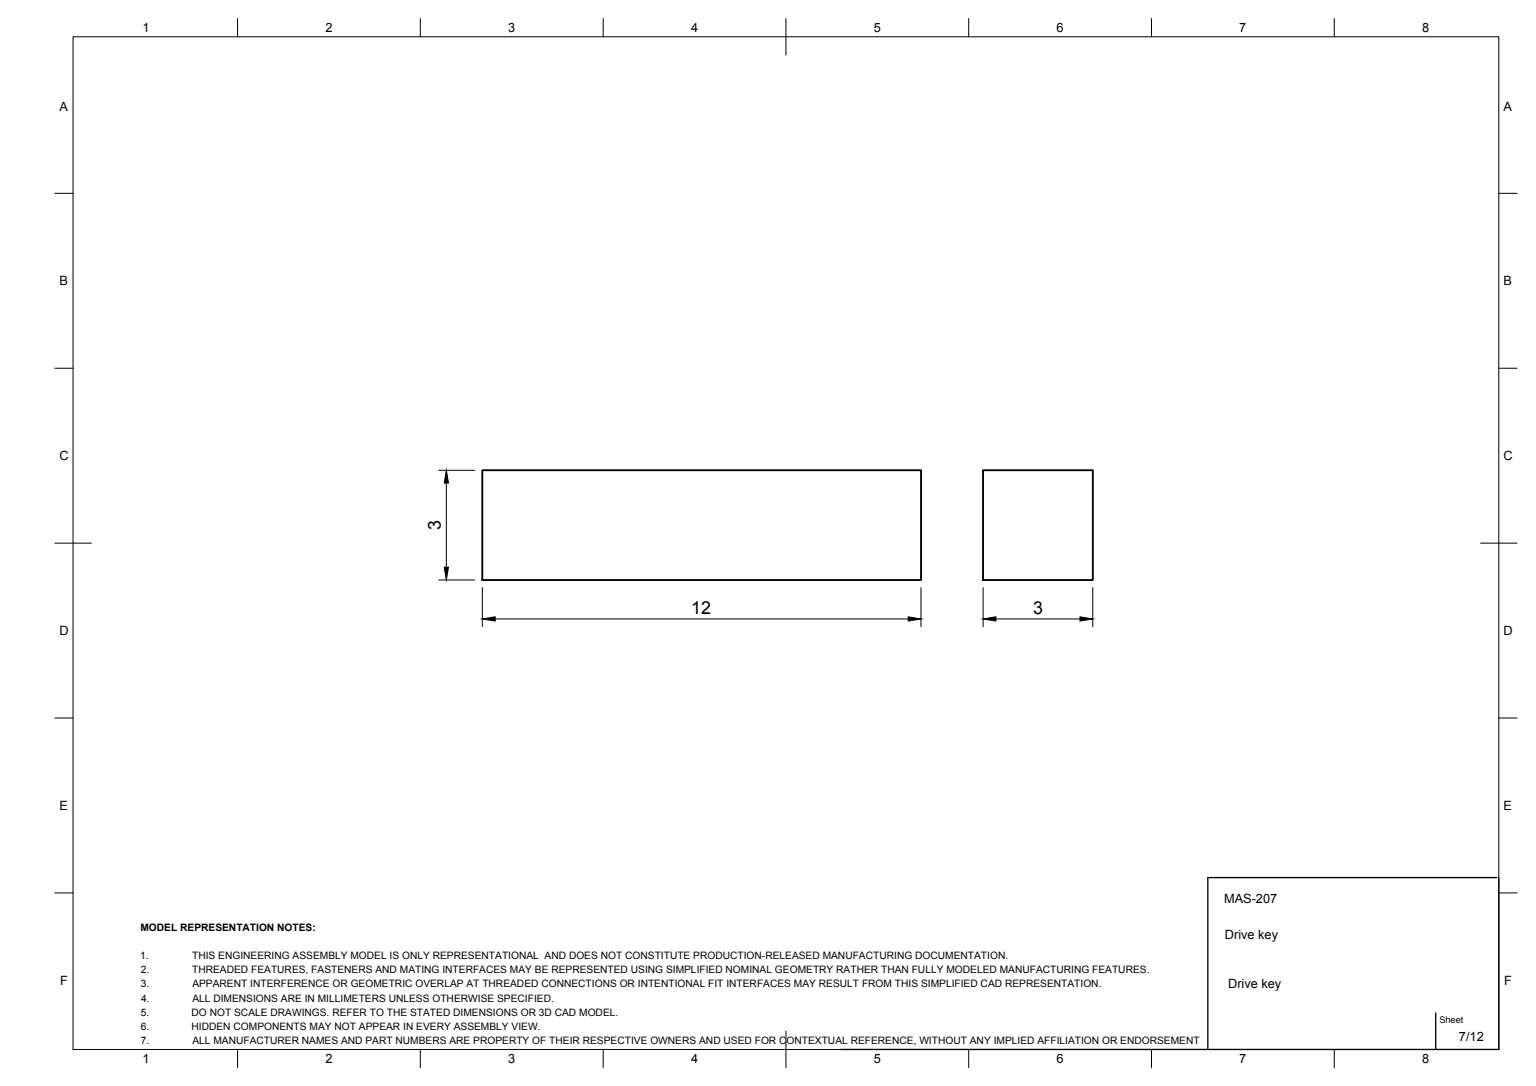
ISO-10303-21;
HEADER;
/* Generated by software containing ST-Developer
 * from STEP Tools, Inc. (www.steptools.com) 
 */

FILE_DESCRIPTION(
/* description */ ('Independent six-slot Geneva indexer. Center distance100, drive radius
50, 60degree indexing per input revolution with120degree engagement an
d240degree dwell. Native machined concave locking faces and relieved d
isk; replaceable retained drive pin; keyed output shaft. Geometry traj
ectory checks use calculated indexing positions, not a contact-dynamic
s simulation. No load or production rating assigned.'),
/* implementation_level */ '2;1');

FILE_NAME(
/* name */ 'Drive key.step',
/* time_stamp */ '2026-11-09T17:53:22-08:00',
/* author */ (''),
/* organization */ (''),
/* preprocessor_version */ 'ST-DEVELOPER v20.2',
/* originating_system */ 'Autodesk Translation Framework v15.17.0.0',
/* authorisation */ '');

FILE_SCHEMA (('AUTOMOTIVE_DESIGN { 1 0 10303 214 3 1 1 }'));
ENDSEC;

DATA;
#10=MECHANICAL_DESIGN_GEOMETRIC_PRESENTATION_REPRESENTATION('',(#105),#4149);
#83=SHAPE_REPRESENTATION_RELATIONSHIP('SRR','None',#4200,#94);
#94=ADVANCED_BREP_SHAPE_REPRESENTATION('',(#116),#4142);
#105=STYLED_ITEM('',(#4264),#116);
#116=MANIFOLD_SOLID_BREP('Body1',#2299);
#213=PLANE('',#2621);
#214=PLANE('',#2622);
#215=PLANE('',#2623);
#216=PLANE('',#2624);
#217=PLANE('',#2625);
#218=PLANE('',#2626);
#333=FACE_OUTER_BOUND('',#494,.T.);
#334=FACE_OUTER_BOUND('',#495,.T.);
#335=FACE_OUTER_BOUND('',#496,.T.);
#336=FACE_OUTER_BOUND('',#497,.T.);
#337=FACE_OUTER_BOUND('',#498,.T.);
#338=FACE_OUTER_BOUND('',#499,.T.);
#494=EDGE_LOOP('',(#1968,#1969,#1970,#1971));
#495=EDGE_LOOP('',(#1972,#1973,#1974,#1975));
#496=EDGE_LOOP('',(#1976,#1977,#1978,#1979));
#497=EDGE_LOOP('',(#1980,#1981,#1982,#1983));
#498=EDGE_LOOP('',(#1984,#1985,#1986,#1987));
#499=EDGE_LOOP('',(#1988,#1989,#1990,#1991));
#686=LINE('',#3953,#858);
#687=LINE('',#3955,#859);
#688=LINE('',#3957,#860);
#689=LINE('',#3958,#861);
#690=LINE('',#3961,#862);
#691=LINE('',#3963,#863);
#692=LINE('',#3964,#864);
#693=LINE('',#3967,#865);
#694=LINE('',#3969,#866);
#695=LINE('',#3970,#867);
#696=LINE('',#3972,#868);
#697=LINE('',#3973,#869);
#858=VECTOR('',#3243,10.);
#859=VECTOR('',#3244,10.);
#860=VECTOR('',#3245,10.);
#861=VECTOR('',#3246,10.);
#862=VECTOR('',#3249,10.);
#863=VECTOR('',#3250,10.);
#864=VECTOR('',#3251,10.);
#865=VECTOR('',#3254,10.);
#866=VECTOR('',#3255,10.);
#867=VECTOR('',#3256,10.);
#868=VECTOR('',#3259,10.);
#869=VECTOR('',#3260,10.);
#1168=VERTEX_POINT('',#3951);
#1169=VERTEX_POINT('',#3952);
#1170=VERTEX_POINT('',#3954);
#1171=VERTEX_POINT('',#3956);
#1172=VERTEX_POINT('',#3960);
#1173=VERTEX_POINT('',#3962);
#1174=VERTEX_POINT('',#3966);
#1175=VERTEX_POINT('',#3968);
#1442=EDGE_CURVE('',#1168,#1169,#686,.T.);
#1443=EDGE_CURVE('',#1169,#1170,#687,.T.);
#1444=EDGE_CURVE('',#1171,#1170,#688,.T.);
#1445=EDGE_CURVE('',#1168,#1171,#689,.T.);
#1446=EDGE_CURVE('',#1172,#1168,#690,.T.);
#1447=EDGE_CURVE('',#1173,#1171,#691,.T.);
#1448=EDGE_CURVE('',#1172,#1173,#692,.T.);
#1449=EDGE_CURVE('',#1174,#1172,#693,.T.);
#1450=EDGE_CURVE('',#1175,#1173,#694,.T.);
#1451=EDGE_CURVE('',#1174,#1175,#695,.T.);
#1452=EDGE_CURVE('',#1169,#1174,#696,.T.);
#1453=EDGE_CURVE('',#1170,#1175,#697,.T.);
#1968=ORIENTED_EDGE('',*,*,#1442,.T.);
#1969=ORIENTED_EDGE('',*,*,#1443,.T.);
#1970=ORIENTED_EDGE('',*,*,#1444,.F.);
#1971=ORIENTED_EDGE('',*,*,#1445,.F.);
#1972=ORIENTED_EDGE('',*,*,#1446,.T.);
#1973=ORIENTED_EDGE('',*,*,#1445,.T.);
#1974=ORIENTED_EDGE('',*,*,#1447,.F.);
#1975=ORIENTED_EDGE('',*,*,#1448,.F.);
#1976=ORIENTED_EDGE('',*,*,#1449,.T.);
#1977=ORIENTED_EDGE('',*,*,#1448,.T.);
#1978=ORIENTED_EDGE('',*,*,#1450,.F.);
#1979=ORIENTED_EDGE('',*,*,#1451,.F.);
#1980=ORIENTED_EDGE('',*,*,#1452,.T.);
#1981=ORIENTED_EDGE('',*,*,#1451,.T.);
#1982=ORIENTED_EDGE('',*,*,#1453,.F.);
#1983=ORIENTED_EDGE('',*,*,#1443,.F.);
#1984=ORIENTED_EDGE('',*,*,#1453,.T.);
#1985=ORIENTED_EDGE('',*,*,#1450,.T.);
#1986=ORIENTED_EDGE('',*,*,#1447,.T.);
#1987=ORIENTED_EDGE('',*,*,#1444,.T.);
#1988=ORIENTED_EDGE('',*,*,#1452,.F.);
#1989=ORIENTED_EDGE('',*,*,#1442,.F.);
#1990=ORIENTED_EDGE('',*,*,#1446,.F.);
#1991=ORIENTED_EDGE('',*,*,#1449,.F.);
#2254=ADVANCED_FACE('',(#333),#213,.T.);
#2255=ADVANCED_FACE('',(#334),#214,.T.);
#2256=ADVANCED_FACE('',(#335),#215,.T.);
#2257=ADVANCED_FACE('',(#336),#216,.T.);
#2258=ADVANCED_FACE('',(#337),#217,.T.);
#2259=ADVANCED_FACE('',(#338),#218,.F.);
#2299=CLOSED_SHELL('',(#2254,#2255,#2256,#2257,#2258,#2259));
#2620=AXIS2_PLACEMENT_3D('',#3949,#3239,#3240);
#2621=AXIS2_PLACEMENT_3D('',#3950,#3241,#3242);
#2622=AXIS2_PLACEMENT_3D('',#3959,#3247,#3248);
#2623=AXIS2_PLACEMENT_3D('',#3965,#3252,#3253);
#2624=AXIS2_PLACEMENT_3D('',#3971,#3257,#3258);
#2625=AXIS2_PLACEMENT_3D('',#3974,#3261,#3262);
#2626=AXIS2_PLACEMENT_3D('',#3975,#3263,#3264);
#3239=DIRECTION('axis',(0.,0.,1.));
#3240=DIRECTION('refdir',(1.,0.,0.));
#3241=DIRECTION('center_axis',(0.,1.,0.));
#3242=DIRECTION('ref_axis',(-1.,0.,0.));
#3243=DIRECTION('',(-1.,0.,0.));
#3244=DIRECTION('',(0.,0.,1.));
#3245=DIRECTION('',(-1.,0.,0.));
#3246=DIRECTION('',(0.,0.,1.));
#3247=DIRECTION('center_axis',(1.,0.,0.));
#3248=DIRECTION('ref_axis',(0.,1.,0.));
#3249=DIRECTION('',(0.,1.,0.));
#3250=DIRECTION('',(0.,1.,0.));
#3251=DIRECTION('',(0.,0.,1.));
#3252=DIRECTION('center_axis',(0.,-1.,0.));
#3253=DIRECTION('ref_axis',(1.,0.,0.));
#3254=DIRECTION('',(1.,0.,0.));
#3255=DIRECTION('',(1.,0.,0.));
#3256=DIRECTION('',(0.,0.,1.));
#3257=DIRECTION('center_axis',(-1.,0.,0.));
#3258=DIRECTION('ref_axis',(0.,-1.,0.));
#3259=DIRECTION('',(0.,-1.,0.));
#3260=DIRECTION('',(0.,-1.,0.));
#3261=DIRECTION('center_axis',(0.,0.,1.));
#3262=DIRECTION('ref_axis',(1.,0.,0.));
#3263=DIRECTION('center_axis',(0.,0.,1.));
#3264=DIRECTION('ref_axis',(1.,0.,0.));
#3949=CARTESIAN_POINT('',(0.,0.,0.));
#3950=CARTESIAN_POINT('Origin',(6.,1.5,32.));
#3951=CARTESIAN_POINT('',(6.,1.5,32.));
#3952=CARTESIAN_POINT('',(3.,1.5,32.));
#3953=CARTESIAN_POINT('',(6.,1.5,32.));
#3954=CARTESIAN_POINT('',(3.,1.5,44.));
#3955=CARTESIAN_POINT('',(3.,1.5,32.));
#3956=CARTESIAN_POINT('',(6.,1.5,44.));
#3957=CARTESIAN_POINT('',(6.,1.5,44.));
#3958=CARTESIAN_POINT('',(6.,1.5,32.));
#3959=CARTESIAN_POINT('Origin',(6.,-1.5,32.));
#3960=CARTESIAN_POINT('',(6.,-1.5,32.));
#3961=CARTESIAN_POINT('',(6.,-1.5,32.));
#3962=CARTESIAN_POINT('',(6.,-1.5,44.));
#3963=CARTESIAN_POINT('',(6.,-1.5,44.));
#3964=CARTESIAN_POINT('',(6.,-1.5,32.));
#3965=CARTESIAN_POINT('Origin',(3.,-1.5,32.));
#3966=CARTESIAN_POINT('',(3.,-1.5,32.));
#3967=CARTESIAN_POINT('',(3.,-1.5,32.));
#3968=CARTESIAN_POINT('',(3.,-1.5,44.));
#3969=CARTESIAN_POINT('',(3.,-1.5,44.));
#3970=CARTESIAN_POINT('',(3.,-1.5,32.));
#3971=CARTESIAN_POINT('Origin',(3.,1.5,32.));
#3972=CARTESIAN_POINT('',(3.,1.5,32.));
#3973=CARTESIAN_POINT('',(3.,1.5,44.));
#3974=CARTESIAN_POINT('Origin',(4.5,0.,44.));
#3975=CARTESIAN_POINT('Origin',(4.5,0.,32.));
#4129=UNCERTAINTY_MEASURE_WITH_UNIT(LENGTH_MEASURE(0.01),#4150,
'DISTANCE_ACCURACY_VALUE',
'Maximum model space distance between geometric entities at asserted c
onnectivities');
#4136=UNCERTAINTY_MEASURE_WITH_UNIT(LENGTH_MEASURE(0.01),#4150,
'DISTANCE_ACCURACY_VALUE',
'Maximum model space distance between geometric entities at asserted c
onnectivities');
#4142=(
GEOMETRIC_REPRESENTATION_CONTEXT(3)
GLOBAL_UNCERTAINTY_ASSIGNED_CONTEXT((#4129))
GLOBAL_UNIT_ASSIGNED_CONTEXT((#4150,#4152,#4153))
REPRESENTATION_CONTEXT('','3D')
);
#4149=(
GEOMETRIC_REPRESENTATION_CONTEXT(3)
GLOBAL_UNCERTAINTY_ASSIGNED_CONTEXT((#4136))
GLOBAL_UNIT_ASSIGNED_CONTEXT((#4150,#4152,#4153))
REPRESENTATION_CONTEXT('','3D')
);
#4150=(
LENGTH_UNIT()
NAMED_UNIT(*)
SI_UNIT(.MILLI.,.METRE.)
);
#4152=(
NAMED_UNIT(*)
PLANE_ANGLE_UNIT()
SI_UNIT($,.RADIAN.)
);
#4153=(
NAMED_UNIT(*)
SI_UNIT($,.STERADIAN.)
SOLID_ANGLE_UNIT()
);
#4159=SHAPE_DEFINITION_REPRESENTATION(#4171,#4200);
#4171=PRODUCT_DEFINITION_SHAPE('',$,#4213);
#4200=SHAPE_REPRESENTATION('',(#2620),#4142);
#4207=PRODUCT_DEFINITION_CONTEXT('part definition',#4245,'design');
#4213=PRODUCT_DEFINITION('Drive key','Drive key',#4225,#4207);
#4225=PRODUCT_DEFINITION_FORMATION('',$,#4252);
#4245=APPLICATION_CONTEXT(
'Core Data for Automotive Mechanical Design Process');
#4246=PRODUCT_CONTEXT('part definition',#4245,'mechanical');
#4252=PRODUCT('Drive key','Drive key',$,(#4246));
#4264=PRESENTATION_STYLE_ASSIGNMENT((#4274));
#4274=SURFACE_STYLE_USAGE(.BOTH.,#4284);
#4284=SURFACE_SIDE_STYLE('',(#4294));
#4294=SURFACE_STYLE_FILL_AREA(#4304);
#4304=FILL_AREA_STYLE('Key gray',(#4314));
#4314=FILL_AREA_STYLE_COLOUR('Key gray',#4324);
#4324=COLOUR_RGB('Key gray',0.725490196078431,0.752941176470588,0.792156862745098);
ENDSEC;
END-ISO-10303-21;
